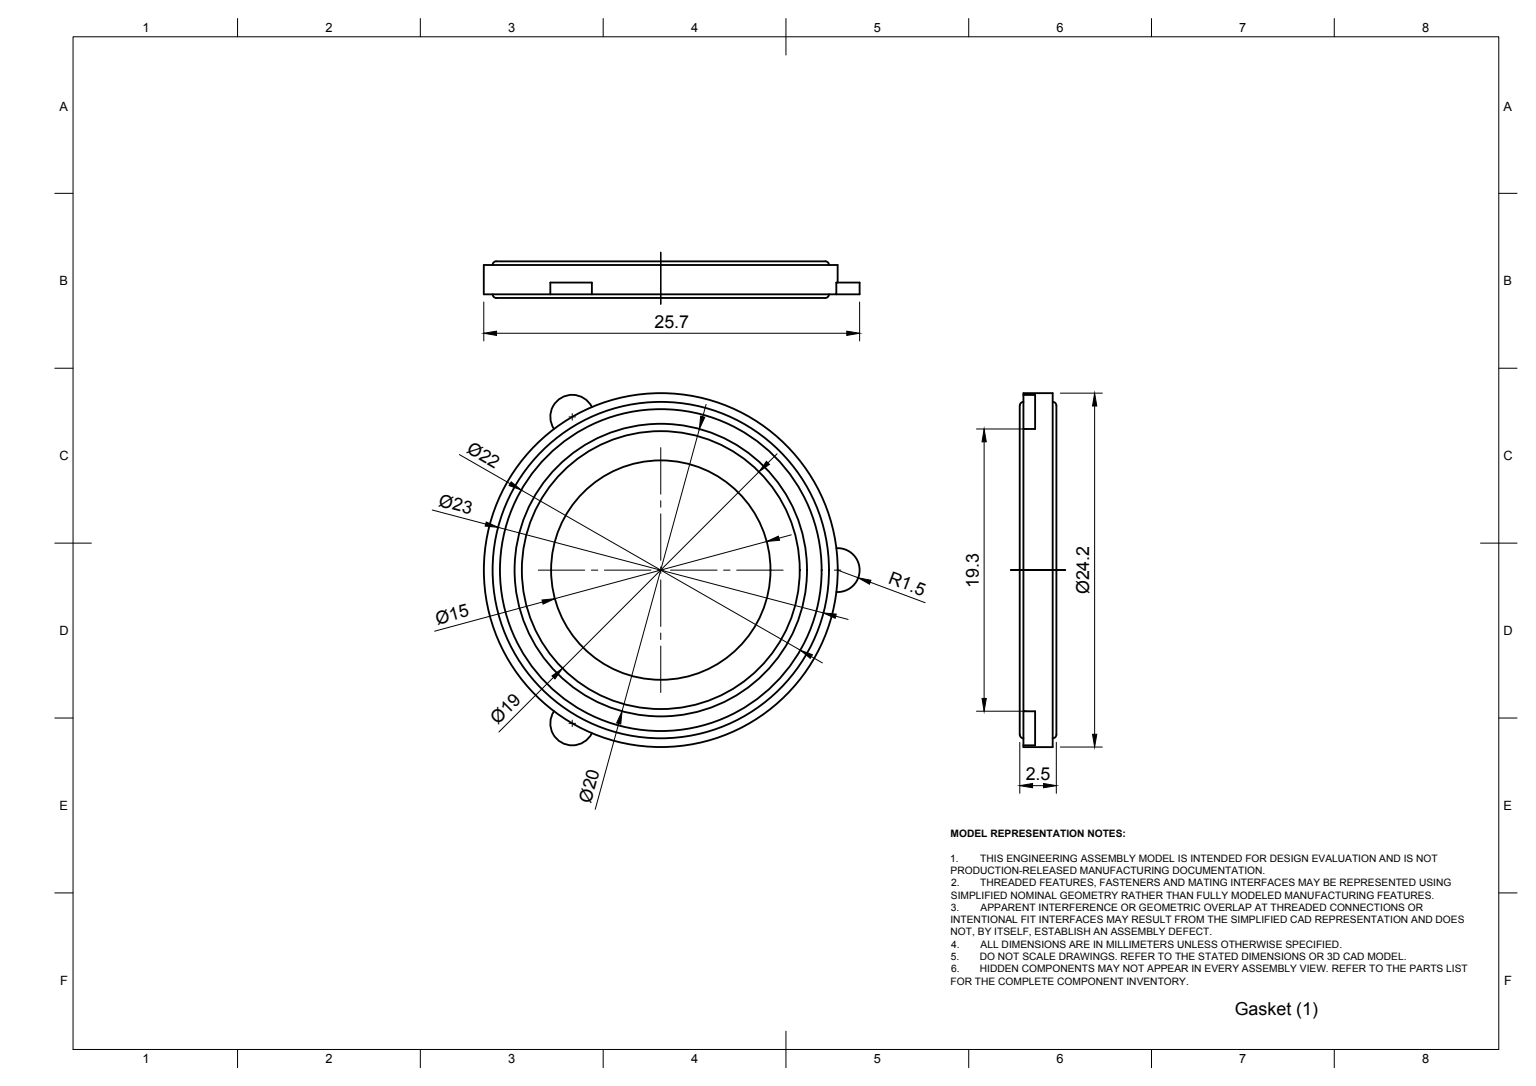
ISO-10303-21;
HEADER;
/* Generated by software containing ST-Developer
 * from STEP Tools, Inc. (www.steptools.com) 
 */

FILE_DESCRIPTION(
/* description */ ('STEP AP214'),
/* implementation_level */ '2;1');

FILE_NAME(
/* name */ 'Gasket (1).step',
/* time_stamp */ '2026-10-05T23:18:41-07:00',
/* author */ (''),
/* organization */ (''),
/* preprocessor_version */ 'ST-DEVELOPER v20.2',
/* originating_system */ 'Autodesk Translation Framework v15.15.0.0',
/* authorisation */ '');

FILE_SCHEMA (('AUTOMOTIVE_DESIGN { 1 0 10303 214 3 1 1 }'));
ENDSEC;

DATA;
#10=MECHANICAL_DESIGN_GEOMETRIC_PRESENTATION_REPRESENTATION('',(#103),#221662);
#65=MANIFOLD_SOLID_BREP('Body1',#79325);
#77=SHAPE_REPRESENTATION_RELATIONSHIP('SRR','None',#221712,#90);
#90=ADVANCED_BREP_SHAPE_REPRESENTATION('',(#65),#221652);
#103=STYLED_ITEM('',(#221783),#65);
#282=FACE_BOUND('',#24733,.T.);
#283=FACE_BOUND('',#24735,.T.);
#284=FACE_BOUND('',#24737,.T.);
#285=FACE_BOUND('',#24739,.T.);
#286=FACE_BOUND('',#24741,.T.);
#287=FACE_BOUND('',#24743,.T.);
#1888=TOROIDAL_SURFACE('',#80621,9.75,0.25);
#1889=TOROIDAL_SURFACE('',#80625,11.25,0.25);
#1890=TOROIDAL_SURFACE('',#80638,11.25,0.25);
#1891=TOROIDAL_SURFACE('',#80642,9.75,0.25);
#2206=CYLINDRICAL_SURFACE('',#80629,12.1);
#2207=CYLINDRICAL_SURFACE('',#80646,7.50000000000001);
#2208=CYLINDRICAL_SURFACE('',#80649,1.5);
#2209=CYLINDRICAL_SURFACE('',#80652,1.5);
#2210=CYLINDRICAL_SURFACE('',#80658,1.5);
#3108=LINE('',#174703,#10175);
#3109=LINE('',#174707,#10176);
#3110=LINE('',#174711,#10177);
#3111=LINE('',#174715,#10178);
#3112=LINE('',#174719,#10179);
#3113=LINE('',#174723,#10180);
#3114=LINE('',#174727,#10181);
#3115=LINE('',#174745,#10182);
#10175=VECTOR('',#88869,12.1);
#10176=VECTOR('',#88872,1000.);
#10177=VECTOR('',#88875,1000.);
#10178=VECTOR('',#88878,1000.);
#10179=VECTOR('',#88881,1000.);
#10180=VECTOR('',#88884,1000.);
#10181=VECTOR('',#88887,1000.);
#10182=VECTOR('',#88910,7.50000000000001);
#16962=PLANE('',#80655);
#16963=PLANE('',#80656);
#16964=PLANE('',#80660);
#16965=PLANE('',#80661);
#16966=PLANE('',#80662);
#16967=PLANE('',#80663);
#16968=PLANE('',#80664);
#16969=PLANE('',#80665);
#16970=PLANE('',#80666);
#20668=FACE_OUTER_BOUND('',#24720,.T.);
#20669=FACE_OUTER_BOUND('',#24721,.T.);
#20670=FACE_OUTER_BOUND('',#24722,.T.);
#20671=FACE_OUTER_BOUND('',#24723,.T.);
#20672=FACE_OUTER_BOUND('',#24724,.T.);
#20673=FACE_OUTER_BOUND('',#24725,.T.);
#20674=FACE_OUTER_BOUND('',#24726,.T.);
#20675=FACE_OUTER_BOUND('',#24727,.T.);
#20676=FACE_OUTER_BOUND('',#24728,.T.);
#20677=FACE_OUTER_BOUND('',#24729,.T.);
#20678=FACE_OUTER_BOUND('',#24730,.T.);
#20679=FACE_OUTER_BOUND('',#24731,.T.);
#20680=FACE_OUTER_BOUND('',#24732,.T.);
#20681=FACE_OUTER_BOUND('',#24734,.T.);
#20682=FACE_OUTER_BOUND('',#24736,.T.);
#20683=FACE_OUTER_BOUND('',#24738,.T.);
#20684=FACE_OUTER_BOUND('',#24740,.T.);
#20685=FACE_OUTER_BOUND('',#24742,.T.);
#24720=EDGE_LOOP('',(#56303,#56304,#56305,#56306));
#24721=EDGE_LOOP('',(#56307,#56308,#56309,#56310));
#24722=EDGE_LOOP('',(#56311,#56312,#56313,#56314,#56315,#56316,#56317,#56318,
#56319,#56320,#56321,#56322,#56323,#56324,#56325,#56326));
#24723=EDGE_LOOP('',(#56327,#56328,#56329,#56330));
#24724=EDGE_LOOP('',(#56331,#56332,#56333,#56334));
#24725=EDGE_LOOP('',(#56335,#56336,#56337,#56338));
#24726=EDGE_LOOP('',(#56339,#56340,#56341,#56342));
#24727=EDGE_LOOP('',(#56343,#56344,#56345,#56346));
#24728=EDGE_LOOP('',(#56347,#56348));
#24729=EDGE_LOOP('',(#56349,#56350));
#24730=EDGE_LOOP('',(#56351,#56352,#56353,#56354));
#24731=EDGE_LOOP('',(#56355,#56356));
#24732=EDGE_LOOP('',(#56357));
#24733=EDGE_LOOP('',(#56358));
#24734=EDGE_LOOP('',(#56359));
#24735=EDGE_LOOP('',(#56360));
#24736=EDGE_LOOP('',(#56361));
#24737=EDGE_LOOP('',(#56362));
#24738=EDGE_LOOP('',(#56363,#56364,#56365,#56366,#56367,#56368,#56369));
#24739=EDGE_LOOP('',(#56370));
#24740=EDGE_LOOP('',(#56371));
#24741=EDGE_LOOP('',(#56372));
#24742=EDGE_LOOP('',(#56373));
#24743=EDGE_LOOP('',(#56374));
#31221=CIRCLE('',#80622,9.49999999999999);
#31222=CIRCLE('',#80623,0.25);
#31223=CIRCLE('',#80624,10.);
#31224=CIRCLE('',#80626,11.);
#31225=CIRCLE('',#80627,0.25);
#31226=CIRCLE('',#80628,11.5);
#31227=CIRCLE('',#80630,12.1);
#31228=CIRCLE('',#80631,12.1);
#31229=CIRCLE('',#80632,12.1);
#31230=CIRCLE('',#80633,12.1);
#31231=CIRCLE('',#80634,12.1);
#31232=CIRCLE('',#80635,12.1);
#31233=CIRCLE('',#80636,12.1);
#31234=CIRCLE('',#80637,12.1);
#31235=CIRCLE('',#80639,11.5);
#31236=CIRCLE('',#80640,0.25);
#31237=CIRCLE('',#80641,11.);
#31238=CIRCLE('',#80643,10.);
#31239=CIRCLE('',#80644,0.25);
#31240=CIRCLE('',#80645,9.49999999999999);
#31241=CIRCLE('',#80647,7.50000000000001);
#31242=CIRCLE('',#80648,7.50000000000001);
#31243=CIRCLE('',#80650,1.5);
#31244=CIRCLE('',#80651,1.5);
#31245=CIRCLE('',#80653,1.49999999999999);
#31246=CIRCLE('',#80654,1.49999999999999);
#31247=CIRCLE('',#80657,1.5);
#31248=CIRCLE('',#80659,1.5);
#34741=VERTEX_POINT('',#174688);
#34742=VERTEX_POINT('',#174690);
#34743=VERTEX_POINT('',#174694);
#34744=VERTEX_POINT('',#174696);
#34745=VERTEX_POINT('',#174700);
#34746=VERTEX_POINT('',#174702);
#34747=VERTEX_POINT('',#174704);
#34748=VERTEX_POINT('',#174706);
#34749=VERTEX_POINT('',#174708);
#34750=VERTEX_POINT('',#174710);
#34751=VERTEX_POINT('',#174712);
#34752=VERTEX_POINT('',#174714);
#34753=VERTEX_POINT('',#174716);
#34754=VERTEX_POINT('',#174718);
#34755=VERTEX_POINT('',#174720);
#34756=VERTEX_POINT('',#174722);
#34757=VERTEX_POINT('',#174724);
#34758=VERTEX_POINT('',#174726);
#34759=VERTEX_POINT('',#174730);
#34760=VERTEX_POINT('',#174732);
#34761=VERTEX_POINT('',#174736);
#34762=VERTEX_POINT('',#174738);
#34763=VERTEX_POINT('',#174742);
#34764=VERTEX_POINT('',#174744);
#42984=EDGE_CURVE('',#34741,#34741,#31221,.T.);
#42985=EDGE_CURVE('',#34741,#34742,#31222,.T.);
#42986=EDGE_CURVE('',#34742,#34742,#31223,.T.);
#42987=EDGE_CURVE('',#34743,#34743,#31224,.T.);
#42988=EDGE_CURVE('',#34743,#34744,#31225,.T.);
#42989=EDGE_CURVE('',#34744,#34744,#31226,.T.);
#42990=EDGE_CURVE('',#34745,#34745,#31227,.T.);
#42991=EDGE_CURVE('',#34745,#34746,#3108,.T.);
#42992=EDGE_CURVE('',#34746,#34747,#31228,.T.);
#42993=EDGE_CURVE('',#34748,#34747,#3109,.T.);
#42994=EDGE_CURVE('',#34748,#34749,#31229,.T.);
#42995=EDGE_CURVE('',#34750,#34749,#3110,.T.);
#42996=EDGE_CURVE('',#34750,#34751,#31230,.T.);
#42997=EDGE_CURVE('',#34752,#34751,#3111,.T.);
#42998=EDGE_CURVE('',#34752,#34753,#31231,.T.);
#42999=EDGE_CURVE('',#34754,#34753,#3112,.T.);
#43000=EDGE_CURVE('',#34754,#34755,#31232,.T.);
#43001=EDGE_CURVE('',#34756,#34755,#3113,.T.);
#43002=EDGE_CURVE('',#34756,#34757,#31233,.T.);
#43003=EDGE_CURVE('',#34758,#34757,#3114,.T.);
#43004=EDGE_CURVE('',#34758,#34746,#31234,.T.);
#43005=EDGE_CURVE('',#34759,#34759,#31235,.T.);
#43006=EDGE_CURVE('',#34759,#34760,#31236,.T.);
#43007=EDGE_CURVE('',#34760,#34760,#31237,.T.);
#43008=EDGE_CURVE('',#34761,#34761,#31238,.T.);
#43009=EDGE_CURVE('',#34761,#34762,#31239,.T.);
#43010=EDGE_CURVE('',#34762,#34762,#31240,.T.);
#43011=EDGE_CURVE('',#34763,#34763,#31241,.T.);
#43012=EDGE_CURVE('',#34763,#34764,#3115,.T.);
#43013=EDGE_CURVE('',#34764,#34764,#31242,.T.);
#43014=EDGE_CURVE('',#34757,#34756,#31243,.T.);
#43015=EDGE_CURVE('',#34758,#34755,#31244,.T.);
#43016=EDGE_CURVE('',#34749,#34748,#31245,.T.);
#43017=EDGE_CURVE('',#34750,#34747,#31246,.T.);
#43018=EDGE_CURVE('',#34753,#34752,#31247,.T.);
#43019=EDGE_CURVE('',#34754,#34751,#31248,.T.);
#56303=ORIENTED_EDGE('',*,*,#42984,.F.);
#56304=ORIENTED_EDGE('',*,*,#42985,.T.);
#56305=ORIENTED_EDGE('',*,*,#42986,.T.);
#56306=ORIENTED_EDGE('',*,*,#42985,.F.);
#56307=ORIENTED_EDGE('',*,*,#42987,.F.);
#56308=ORIENTED_EDGE('',*,*,#42988,.T.);
#56309=ORIENTED_EDGE('',*,*,#42989,.T.);
#56310=ORIENTED_EDGE('',*,*,#42988,.F.);
#56311=ORIENTED_EDGE('',*,*,#42990,.F.);
#56312=ORIENTED_EDGE('',*,*,#42991,.T.);
#56313=ORIENTED_EDGE('',*,*,#42992,.T.);
#56314=ORIENTED_EDGE('',*,*,#42993,.F.);
#56315=ORIENTED_EDGE('',*,*,#42994,.T.);
#56316=ORIENTED_EDGE('',*,*,#42995,.F.);
#56317=ORIENTED_EDGE('',*,*,#42996,.T.);
#56318=ORIENTED_EDGE('',*,*,#42997,.F.);
#56319=ORIENTED_EDGE('',*,*,#42998,.T.);
#56320=ORIENTED_EDGE('',*,*,#42999,.F.);
#56321=ORIENTED_EDGE('',*,*,#43000,.T.);
#56322=ORIENTED_EDGE('',*,*,#43001,.F.);
#56323=ORIENTED_EDGE('',*,*,#43002,.T.);
#56324=ORIENTED_EDGE('',*,*,#43003,.F.);
#56325=ORIENTED_EDGE('',*,*,#43004,.T.);
#56326=ORIENTED_EDGE('',*,*,#42991,.F.);
#56327=ORIENTED_EDGE('',*,*,#43005,.F.);
#56328=ORIENTED_EDGE('',*,*,#43006,.T.);
#56329=ORIENTED_EDGE('',*,*,#43007,.T.);
#56330=ORIENTED_EDGE('',*,*,#43006,.F.);
#56331=ORIENTED_EDGE('',*,*,#43008,.F.);
#56332=ORIENTED_EDGE('',*,*,#43009,.T.);
#56333=ORIENTED_EDGE('',*,*,#43010,.T.);
#56334=ORIENTED_EDGE('',*,*,#43009,.F.);
#56335=ORIENTED_EDGE('',*,*,#43011,.F.);
#56336=ORIENTED_EDGE('',*,*,#43012,.T.);
#56337=ORIENTED_EDGE('',*,*,#43013,.T.);
#56338=ORIENTED_EDGE('',*,*,#43012,.F.);
#56339=ORIENTED_EDGE('',*,*,#43014,.T.);
#56340=ORIENTED_EDGE('',*,*,#43001,.T.);
#56341=ORIENTED_EDGE('',*,*,#43015,.F.);
#56342=ORIENTED_EDGE('',*,*,#43003,.T.);
#56343=ORIENTED_EDGE('',*,*,#43016,.T.);
#56344=ORIENTED_EDGE('',*,*,#42993,.T.);
#56345=ORIENTED_EDGE('',*,*,#43017,.F.);
#56346=ORIENTED_EDGE('',*,*,#42995,.T.);
#56347=ORIENTED_EDGE('',*,*,#42994,.F.);
#56348=ORIENTED_EDGE('',*,*,#43016,.F.);
#56349=ORIENTED_EDGE('',*,*,#42998,.F.);
#56350=ORIENTED_EDGE('',*,*,#43018,.F.);
#56351=ORIENTED_EDGE('',*,*,#43019,.F.);
#56352=ORIENTED_EDGE('',*,*,#42999,.T.);
#56353=ORIENTED_EDGE('',*,*,#43018,.T.);
#56354=ORIENTED_EDGE('',*,*,#42997,.T.);
#56355=ORIENTED_EDGE('',*,*,#43002,.F.);
#56356=ORIENTED_EDGE('',*,*,#43014,.F.);
#56357=ORIENTED_EDGE('',*,*,#42984,.T.);
#56358=ORIENTED_EDGE('',*,*,#43013,.F.);
#56359=ORIENTED_EDGE('',*,*,#43010,.F.);
#56360=ORIENTED_EDGE('',*,*,#43011,.T.);
#56361=ORIENTED_EDGE('',*,*,#43007,.F.);
#56362=ORIENTED_EDGE('',*,*,#43008,.T.);
#56363=ORIENTED_EDGE('',*,*,#42996,.F.);
#56364=ORIENTED_EDGE('',*,*,#43017,.T.);
#56365=ORIENTED_EDGE('',*,*,#42992,.F.);
#56366=ORIENTED_EDGE('',*,*,#43004,.F.);
#56367=ORIENTED_EDGE('',*,*,#43015,.T.);
#56368=ORIENTED_EDGE('',*,*,#43000,.F.);
#56369=ORIENTED_EDGE('',*,*,#43019,.T.);
#56370=ORIENTED_EDGE('',*,*,#43005,.T.);
#56371=ORIENTED_EDGE('',*,*,#42990,.T.);
#56372=ORIENTED_EDGE('',*,*,#42989,.F.);
#56373=ORIENTED_EDGE('',*,*,#42987,.T.);
#56374=ORIENTED_EDGE('',*,*,#42986,.F.);
#76098=ADVANCED_FACE('',(#20668),#1888,.T.);
#76099=ADVANCED_FACE('',(#20669),#1889,.T.);
#76100=ADVANCED_FACE('',(#20670),#2206,.T.);
#76101=ADVANCED_FACE('',(#20671),#1890,.T.);
#76102=ADVANCED_FACE('',(#20672),#1891,.T.);
#76103=ADVANCED_FACE('',(#20673),#2207,.F.);
#76104=ADVANCED_FACE('',(#20674),#2208,.T.);
#76105=ADVANCED_FACE('',(#20675),#2209,.T.);
#76106=ADVANCED_FACE('',(#20676),#16962,.F.);
#76107=ADVANCED_FACE('',(#20677),#16963,.F.);
#76108=ADVANCED_FACE('',(#20678),#2210,.T.);
#76109=ADVANCED_FACE('',(#20679),#16964,.F.);
#76110=ADVANCED_FACE('',(#20680,#282),#16965,.T.);
#76111=ADVANCED_FACE('',(#20681,#283),#16966,.T.);
#76112=ADVANCED_FACE('',(#20682,#284),#16967,.T.);
#76113=ADVANCED_FACE('',(#20683,#285),#16968,.T.);
#76114=ADVANCED_FACE('',(#20684,#286),#16969,.T.);
#76115=ADVANCED_FACE('',(#20685,#287),#16970,.T.);
#79325=CLOSED_SHELL('',(#76098,#76099,#76100,#76101,#76102,#76103,#76104,
#76105,#76106,#76107,#76108,#76109,#76110,#76111,#76112,#76113,#76114,#76115));
#80620=AXIS2_PLACEMENT_3D('',#174686,#88847,#88848);
#80621=AXIS2_PLACEMENT_3D('',#174687,#88849,#88850);
#80622=AXIS2_PLACEMENT_3D('',#174689,#88851,#88852);
#80623=AXIS2_PLACEMENT_3D('',#174691,#88853,#88854);
#80624=AXIS2_PLACEMENT_3D('',#174692,#88855,#88856);
#80625=AXIS2_PLACEMENT_3D('',#174693,#88857,#88858);
#80626=AXIS2_PLACEMENT_3D('',#174695,#88859,#88860);
#80627=AXIS2_PLACEMENT_3D('',#174697,#88861,#88862);
#80628=AXIS2_PLACEMENT_3D('',#174698,#88863,#88864);
#80629=AXIS2_PLACEMENT_3D('',#174699,#88865,#88866);
#80630=AXIS2_PLACEMENT_3D('',#174701,#88867,#88868);
#80631=AXIS2_PLACEMENT_3D('',#174705,#88870,#88871);
#80632=AXIS2_PLACEMENT_3D('',#174709,#88873,#88874);
#80633=AXIS2_PLACEMENT_3D('',#174713,#88876,#88877);
#80634=AXIS2_PLACEMENT_3D('',#174717,#88879,#88880);
#80635=AXIS2_PLACEMENT_3D('',#174721,#88882,#88883);
#80636=AXIS2_PLACEMENT_3D('',#174725,#88885,#88886);
#80637=AXIS2_PLACEMENT_3D('',#174728,#88888,#88889);
#80638=AXIS2_PLACEMENT_3D('',#174729,#88890,#88891);
#80639=AXIS2_PLACEMENT_3D('',#174731,#88892,#88893);
#80640=AXIS2_PLACEMENT_3D('',#174733,#88894,#88895);
#80641=AXIS2_PLACEMENT_3D('',#174734,#88896,#88897);
#80642=AXIS2_PLACEMENT_3D('',#174735,#88898,#88899);
#80643=AXIS2_PLACEMENT_3D('',#174737,#88900,#88901);
#80644=AXIS2_PLACEMENT_3D('',#174739,#88902,#88903);
#80645=AXIS2_PLACEMENT_3D('',#174740,#88904,#88905);
#80646=AXIS2_PLACEMENT_3D('',#174741,#88906,#88907);
#80647=AXIS2_PLACEMENT_3D('',#174743,#88908,#88909);
#80648=AXIS2_PLACEMENT_3D('',#174746,#88911,#88912);
#80649=AXIS2_PLACEMENT_3D('',#174747,#88913,#88914);
#80650=AXIS2_PLACEMENT_3D('',#174748,#88915,#88916);
#80651=AXIS2_PLACEMENT_3D('',#174749,#88917,#88918);
#80652=AXIS2_PLACEMENT_3D('',#174750,#88919,#88920);
#80653=AXIS2_PLACEMENT_3D('',#174751,#88921,#88922);
#80654=AXIS2_PLACEMENT_3D('',#174752,#88923,#88924);
#80655=AXIS2_PLACEMENT_3D('',#174753,#88925,#88926);
#80656=AXIS2_PLACEMENT_3D('',#174754,#88927,#88928);
#80657=AXIS2_PLACEMENT_3D('',#174755,#88929,#88930);
#80658=AXIS2_PLACEMENT_3D('',#174756,#88931,#88932);
#80659=AXIS2_PLACEMENT_3D('',#174757,#88933,#88934);
#80660=AXIS2_PLACEMENT_3D('',#174758,#88935,#88936);
#80661=AXIS2_PLACEMENT_3D('',#174759,#88937,#88938);
#80662=AXIS2_PLACEMENT_3D('',#174760,#88939,#88940);
#80663=AXIS2_PLACEMENT_3D('',#174761,#88941,#88942);
#80664=AXIS2_PLACEMENT_3D('',#174762,#88943,#88944);
#80665=AXIS2_PLACEMENT_3D('',#174763,#88945,#88946);
#80666=AXIS2_PLACEMENT_3D('',#174764,#88947,#88948);
#88847=DIRECTION('axis',(0.,0.,1.));
#88848=DIRECTION('refdir',(1.,0.,0.));
#88849=DIRECTION('center_axis',(1.,0.,0.));
#88850=DIRECTION('ref_axis',(0.,0.,-1.));
#88851=DIRECTION('center_axis',(1.,0.,0.));
#88852=DIRECTION('ref_axis',(0.,0.,-1.));
#88853=DIRECTION('center_axis',(0.,-1.,0.));
#88854=DIRECTION('ref_axis',(0.,0.,1.));
#88855=DIRECTION('center_axis',(1.,0.,0.));
#88856=DIRECTION('ref_axis',(0.,0.,-1.));
#88857=DIRECTION('center_axis',(1.,0.,0.));
#88858=DIRECTION('ref_axis',(0.,0.,-1.));
#88859=DIRECTION('center_axis',(1.,0.,0.));
#88860=DIRECTION('ref_axis',(0.,0.,-1.));
#88861=DIRECTION('center_axis',(0.,-1.,0.));
#88862=DIRECTION('ref_axis',(0.,0.,1.));
#88863=DIRECTION('center_axis',(1.,0.,0.));
#88864=DIRECTION('ref_axis',(0.,0.,-1.));
#88865=DIRECTION('center_axis',(1.,0.,0.));
#88866=DIRECTION('ref_axis',(0.,0.,-1.));
#88867=DIRECTION('center_axis',(1.,0.,0.));
#88868=DIRECTION('ref_axis',(0.,0.,-1.));
#88869=DIRECTION('',(-1.,0.,0.));
#88870=DIRECTION('center_axis',(1.,0.,0.));
#88871=DIRECTION('ref_axis',(0.,0.,-1.));
#88872=DIRECTION('',(-1.,0.,0.));
#88873=DIRECTION('center_axis',(1.,0.,0.));
#88874=DIRECTION('ref_axis',(0.,0.,1.));
#88875=DIRECTION('',(1.,0.,0.));
#88876=DIRECTION('center_axis',(1.,0.,0.));
#88877=DIRECTION('ref_axis',(0.,0.,-1.));
#88878=DIRECTION('',(-1.,0.,0.));
#88879=DIRECTION('center_axis',(1.,0.,0.));
#88880=DIRECTION('ref_axis',(0.,0.,1.));
#88881=DIRECTION('',(1.,0.,0.));
#88882=DIRECTION('center_axis',(1.,0.,0.));
#88883=DIRECTION('ref_axis',(0.,0.,-1.));
#88884=DIRECTION('',(-1.,0.,0.));
#88885=DIRECTION('center_axis',(1.,0.,0.));
#88886=DIRECTION('ref_axis',(0.,0.,1.));
#88887=DIRECTION('',(1.,0.,0.));
#88888=DIRECTION('center_axis',(1.,0.,0.));
#88889=DIRECTION('ref_axis',(0.,0.,-1.));
#88890=DIRECTION('center_axis',(1.,0.,0.));
#88891=DIRECTION('ref_axis',(0.,0.,-1.));
#88892=DIRECTION('center_axis',(1.,0.,0.));
#88893=DIRECTION('ref_axis',(0.,0.,-1.));
#88894=DIRECTION('center_axis',(0.,-1.,0.));
#88895=DIRECTION('ref_axis',(0.,0.,1.));
#88896=DIRECTION('center_axis',(1.,0.,0.));
#88897=DIRECTION('ref_axis',(0.,0.,-1.));
#88898=DIRECTION('center_axis',(1.,0.,0.));
#88899=DIRECTION('ref_axis',(0.,0.,-1.));
#88900=DIRECTION('center_axis',(1.,0.,0.));
#88901=DIRECTION('ref_axis',(0.,0.,-1.));
#88902=DIRECTION('center_axis',(0.,-1.,0.));
#88903=DIRECTION('ref_axis',(0.,0.,1.));
#88904=DIRECTION('center_axis',(1.,0.,0.));
#88905=DIRECTION('ref_axis',(0.,0.,-1.));
#88906=DIRECTION('center_axis',(1.,0.,0.));
#88907=DIRECTION('ref_axis',(0.,0.,-1.));
#88908=DIRECTION('center_axis',(1.,0.,0.));
#88909=DIRECTION('ref_axis',(0.,0.,-1.));
#88910=DIRECTION('',(1.,0.,0.));
#88911=DIRECTION('center_axis',(1.,0.,0.));
#88912=DIRECTION('ref_axis',(0.,0.,-1.));
#88913=DIRECTION('center_axis',(-1.,0.,0.));
#88914=DIRECTION('ref_axis',(0.,1.,-2.82534752406804E-15));
#88915=DIRECTION('center_axis',(-1.,0.,0.));
#88916=DIRECTION('ref_axis',(0.,1.,0.));
#88917=DIRECTION('center_axis',(-1.,0.,0.));
#88918=DIRECTION('ref_axis',(0.,1.,0.));
#88919=DIRECTION('center_axis',(-1.,0.,0.));
#88920=DIRECTION('ref_axis',(0.,0.,1.));
#88921=DIRECTION('center_axis',(-1.,0.,0.));
#88922=DIRECTION('ref_axis',(0.,-0.500000000000002,0.866025403784437));
#88923=DIRECTION('center_axis',(-1.,0.,0.));
#88924=DIRECTION('ref_axis',(0.,-0.500000000000002,0.866025403784437));
#88925=DIRECTION('center_axis',(-1.,0.,0.));
#88926=DIRECTION('ref_axis',(0.,0.,1.));
#88927=DIRECTION('center_axis',(-1.,0.,0.));
#88928=DIRECTION('ref_axis',(0.,0.,1.));
#88929=DIRECTION('center_axis',(-1.,0.,0.));
#88930=DIRECTION('ref_axis',(0.,-0.500000000000001,-0.866025403784438));
#88931=DIRECTION('center_axis',(-1.,0.,0.));
#88932=DIRECTION('ref_axis',(0.,-0.500000000000002,-0.866025403784437));
#88933=DIRECTION('center_axis',(-1.,0.,0.));
#88934=DIRECTION('ref_axis',(0.,-0.500000000000001,-0.866025403784438));
#88935=DIRECTION('center_axis',(-1.,0.,0.));
#88936=DIRECTION('ref_axis',(0.,0.,1.));
#88937=DIRECTION('center_axis',(1.,0.,0.));
#88938=DIRECTION('ref_axis',(0.,1.,0.));
#88939=DIRECTION('center_axis',(-1.,0.,0.));
#88940=DIRECTION('ref_axis',(0.,0.,1.));
#88941=DIRECTION('center_axis',(-1.,0.,0.));
#88942=DIRECTION('ref_axis',(0.,0.,1.));
#88943=DIRECTION('center_axis',(-1.,0.,0.));
#88944=DIRECTION('ref_axis',(0.,0.,1.));
#88945=DIRECTION('center_axis',(1.,0.,0.));
#88946=DIRECTION('ref_axis',(0.,1.,0.));
#88947=DIRECTION('center_axis',(1.,0.,0.));
#88948=DIRECTION('ref_axis',(0.,1.,0.));
#174686=CARTESIAN_POINT('',(0.,0.,0.));
#174687=CARTESIAN_POINT('Origin',(-20.5675364832709,-75.,72.98888938658));
#174688=CARTESIAN_POINT('',(-20.5675364832709,-75.,82.48888938658));
#174689=CARTESIAN_POINT('Origin',(-20.5675364832709,-75.,72.98888938658));
#174690=CARTESIAN_POINT('',(-20.5675364832709,-75.,82.98888938658));
#174691=CARTESIAN_POINT('Origin',(-20.5675364832709,-75.,82.73888938658));
#174692=CARTESIAN_POINT('Origin',(-20.5675364832709,-75.,72.98888938658));
#174693=CARTESIAN_POINT('Origin',(-20.5675364832709,-75.,72.98888938658));
#174694=CARTESIAN_POINT('',(-20.5675364832709,-75.,83.98888938658));
#174695=CARTESIAN_POINT('Origin',(-20.5675364832709,-75.,72.98888938658));
#174696=CARTESIAN_POINT('',(-20.5675364832709,-75.,84.48888938658));
#174697=CARTESIAN_POINT('Origin',(-20.5675364832709,-75.,84.23888938658));
#174698=CARTESIAN_POINT('Origin',(-20.5675364832709,-75.,72.98888938658));
#174699=CARTESIAN_POINT('Origin',(-25.5675364832709,-75.,72.98888938658));
#174700=CARTESIAN_POINT('',(-20.5675364832709,-75.,85.08888938658));
#174701=CARTESIAN_POINT('Origin',(-20.5675364832709,-75.,72.98888938658));
#174702=CARTESIAN_POINT('',(-22.5675364832709,-75.,85.08888938658));
#174703=CARTESIAN_POINT('',(-25.5675364832709,-75.,85.08888938658));
#174704=CARTESIAN_POINT('',(-22.5675364832709,-79.7069721126241,84.1358357635471));
#174705=CARTESIAN_POINT('Origin',(-22.5675364832709,-75.,72.98888938658));
#174706=CARTESIAN_POINT('',(-21.7675364832709,-79.7069721126241,84.1358357635471));
#174707=CARTESIAN_POINT('',(-22.1675364832709,-79.7069721126241,84.1358357635471));
#174708=CARTESIAN_POINT('',(-21.7675364832709,-82.3000526807644,82.6387199995009));
#174709=CARTESIAN_POINT('Origin',(-21.7675364832709,-75.,72.98888938658));
#174710=CARTESIAN_POINT('',(-22.5675364832709,-82.3000526807644,82.6387199995009));
#174711=CARTESIAN_POINT('',(-22.1675364832709,-82.3000526807644,82.6387199995009));
#174712=CARTESIAN_POINT('',(-22.5675364832709,-82.3000526807644,63.3390587736591));
#174713=CARTESIAN_POINT('Origin',(-22.5675364832709,-75.,72.98888938658));
#174714=CARTESIAN_POINT('',(-21.7675364832709,-82.3000526807644,63.3390587736591));
#174715=CARTESIAN_POINT('',(-22.1675364832709,-82.3000526807644,63.3390587736591));
#174716=CARTESIAN_POINT('',(-21.7675364832709,-79.7069721126241,61.8419430096129));
#174717=CARTESIAN_POINT('Origin',(-21.7675364832709,-75.,72.98888938658));
#174718=CARTESIAN_POINT('',(-22.5675364832709,-79.7069721126241,61.8419430096129));
#174719=CARTESIAN_POINT('',(-22.1675364832709,-79.7069721126241,61.8419430096129));
#174720=CARTESIAN_POINT('',(-22.5675364832709,-62.9929752066116,71.4917736225339));
#174721=CARTESIAN_POINT('Origin',(-22.5675364832709,-75.,72.98888938658));
#174722=CARTESIAN_POINT('',(-21.7675364832709,-62.9929752066116,71.4917736225339));
#174723=CARTESIAN_POINT('',(-22.1675364832709,-62.9929752066116,71.4917736225339));
#174724=CARTESIAN_POINT('',(-21.7675364832709,-62.9929752066116,74.4860051506262));
#174725=CARTESIAN_POINT('Origin',(-21.7675364832709,-75.,72.98888938658));
#174726=CARTESIAN_POINT('',(-22.5675364832709,-62.9929752066116,74.4860051506262));
#174727=CARTESIAN_POINT('',(-22.1675364832709,-62.9929752066116,74.4860051506262));
#174728=CARTESIAN_POINT('Origin',(-22.5675364832709,-75.,72.98888938658));
#174729=CARTESIAN_POINT('Origin',(-22.5675364832709,-75.,72.98888938658));
#174730=CARTESIAN_POINT('',(-22.5675364832709,-75.,84.48888938658));
#174731=CARTESIAN_POINT('Origin',(-22.5675364832709,-75.,72.98888938658));
#174732=CARTESIAN_POINT('',(-22.5675364832709,-75.,83.98888938658));
#174733=CARTESIAN_POINT('Origin',(-22.5675364832709,-75.,84.23888938658));
#174734=CARTESIAN_POINT('Origin',(-22.5675364832709,-75.,72.98888938658));
#174735=CARTESIAN_POINT('Origin',(-22.5675364832709,-75.,72.98888938658));
#174736=CARTESIAN_POINT('',(-22.5675364832709,-75.,82.98888938658));
#174737=CARTESIAN_POINT('Origin',(-22.5675364832709,-75.,72.98888938658));
#174738=CARTESIAN_POINT('',(-22.5675364832709,-75.,82.48888938658));
#174739=CARTESIAN_POINT('Origin',(-22.5675364832709,-75.,82.73888938658));
#174740=CARTESIAN_POINT('Origin',(-22.5675364832709,-75.,72.98888938658));
#174741=CARTESIAN_POINT('Origin',(-25.5675364832709,-75.,72.98888938658));
#174742=CARTESIAN_POINT('',(-22.5675364832709,-75.,80.48888938658));
#174743=CARTESIAN_POINT('Origin',(-22.5675364832709,-75.,72.98888938658));
#174744=CARTESIAN_POINT('',(-20.5675364832709,-75.,80.48888938658));
#174745=CARTESIAN_POINT('',(-25.5675364832709,-75.,80.48888938658));
#174746=CARTESIAN_POINT('Origin',(-20.5675364832709,-75.,72.98888938658));
#174747=CARTESIAN_POINT('Origin',(-21.7675364832709,-62.9,72.98888938658));
#174748=CARTESIAN_POINT('Origin',(-21.7675364832709,-62.9,72.98888938658));
#174749=CARTESIAN_POINT('Origin',(-22.5675364832709,-62.9,72.98888938658));
#174750=CARTESIAN_POINT('Origin',(-21.7675364832709,-81.05,83.4677967723717));
#174751=CARTESIAN_POINT('Origin',(-21.7675364832709,-81.05,83.4677967723717));
#174752=CARTESIAN_POINT('Origin',(-22.5675364832709,-81.05,83.4677967723717));
#174753=CARTESIAN_POINT('Origin',(-21.7675364832709,-81.05,83.4677967723717));
#174754=CARTESIAN_POINT('Origin',(-21.7675364832709,-81.05,62.5099820007883));
#174755=CARTESIAN_POINT('Origin',(-21.7675364832709,-81.05,62.5099820007883));
#174756=CARTESIAN_POINT('Origin',(-21.7675364832709,-81.05,62.5099820007883));
#174757=CARTESIAN_POINT('Origin',(-22.5675364832709,-81.05,62.5099820007883));
#174758=CARTESIAN_POINT('Origin',(-21.7675364832709,-62.9,72.98888938658));
#174759=CARTESIAN_POINT('Origin',(-20.5675364832709,-82.5,72.98888938658));
#174760=CARTESIAN_POINT('Origin',(-22.5675364832709,-84.5,72.98888938658));
#174761=CARTESIAN_POINT('Origin',(-22.5675364832709,-86.,72.98888938658));
#174762=CARTESIAN_POINT('Origin',(-22.5675364832709,-87.1,72.98888938658));
#174763=CARTESIAN_POINT('Origin',(-20.5675364832709,-86.5,72.98888938658));
#174764=CARTESIAN_POINT('Origin',(-20.5675364832709,-85.,72.98888938658));
#221637=UNCERTAINTY_MEASURE_WITH_UNIT(LENGTH_MEASURE(0.01),#221663,
'DISTANCE_ACCURACY_VALUE',
'Maximum model space distance between geometric entities at asserted c
onnectivities');
#221647=UNCERTAINTY_MEASURE_WITH_UNIT(LENGTH_MEASURE(0.01),#221663,
'DISTANCE_ACCURACY_VALUE',
'Maximum model space distance between geometric entities at asserted c
onnectivities');
#221652=(
GEOMETRIC_REPRESENTATION_CONTEXT(3)
GLOBAL_UNCERTAINTY_ASSIGNED_CONTEXT((#221637))
GLOBAL_UNIT_ASSIGNED_CONTEXT((#221663,#221665,#221666))
REPRESENTATION_CONTEXT('','3D')
);
#221662=(
GEOMETRIC_REPRESENTATION_CONTEXT(3)
GLOBAL_UNCERTAINTY_ASSIGNED_CONTEXT((#221647))
GLOBAL_UNIT_ASSIGNED_CONTEXT((#221663,#221665,#221666))
REPRESENTATION_CONTEXT('','3D')
);
#221663=(
LENGTH_UNIT()
NAMED_UNIT(*)
SI_UNIT(.MILLI.,.METRE.)
);
#221665=(
NAMED_UNIT(*)
PLANE_ANGLE_UNIT()
SI_UNIT($,.RADIAN.)
);
#221666=(
NAMED_UNIT(*)
SI_UNIT($,.STERADIAN.)
SOLID_ANGLE_UNIT()
);
#221671=SHAPE_DEFINITION_REPRESENTATION(#221685,#221712);
#221685=PRODUCT_DEFINITION_SHAPE('',$,#221727);
#221712=SHAPE_REPRESENTATION('',(#80620),#221652);
#221722=PRODUCT_DEFINITION_CONTEXT('part definition',#221766,'design');
#221727=PRODUCT_DEFINITION('2026-10-05-23-02-32-151','Gasket (1)',#221741,
#221722);
#221741=PRODUCT_DEFINITION_FORMATION('',$,#221772);
#221766=APPLICATION_CONTEXT(
'Core Data for Automotive Mechanical Design Process');
#221767=PRODUCT_CONTEXT('part definition',#221766,'mechanical');
#221772=PRODUCT('2026-10-05-23-02-32-151','Gasket (1)',$,(#221767));
#221783=PRESENTATION_STYLE_ASSIGNMENT((#221785));
#221785=SURFACE_STYLE_USAGE(.BOTH.,#221787);
#221787=SURFACE_SIDE_STYLE('',(#221789));
#221789=SURFACE_STYLE_FILL_AREA(#221791);
#221791=FILL_AREA_STYLE('Opaque(202,209,238)',(#221793));
#221793=FILL_AREA_STYLE_COLOUR('Opaque(202,209,238)',#221795);
#221795=COLOUR_RGB('Opaque(202,209,238)', 0.09019608, 0.27058824, 0.51372549);
ENDSEC;
END-ISO-10303-21;
